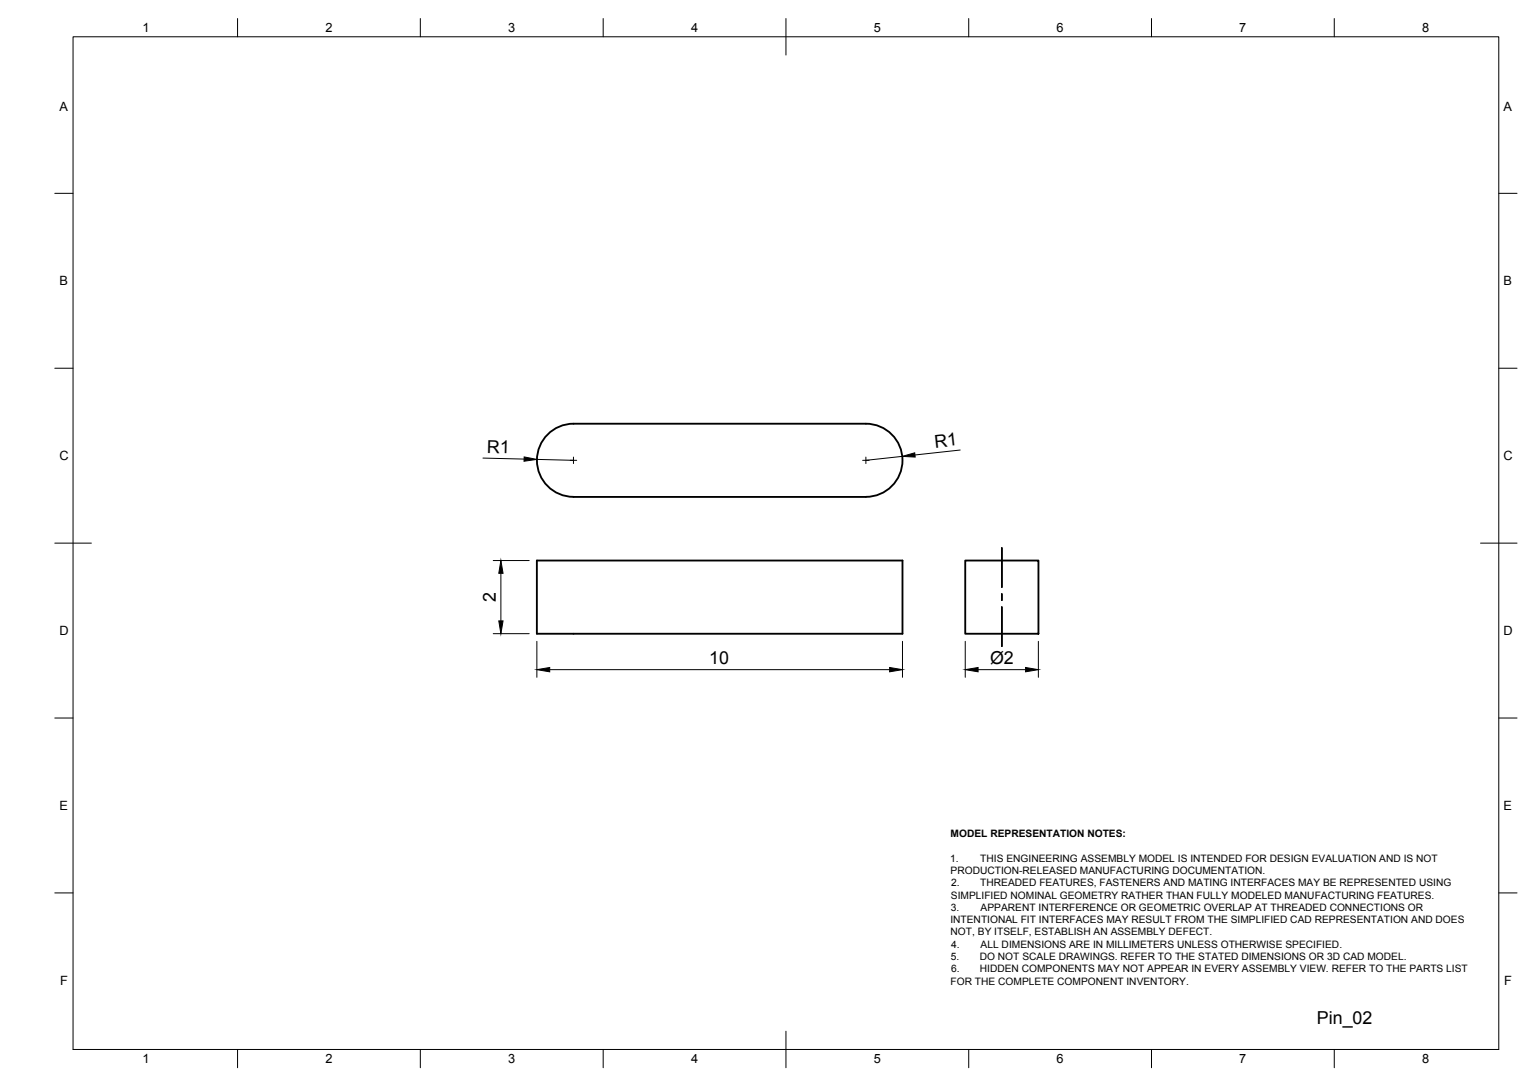
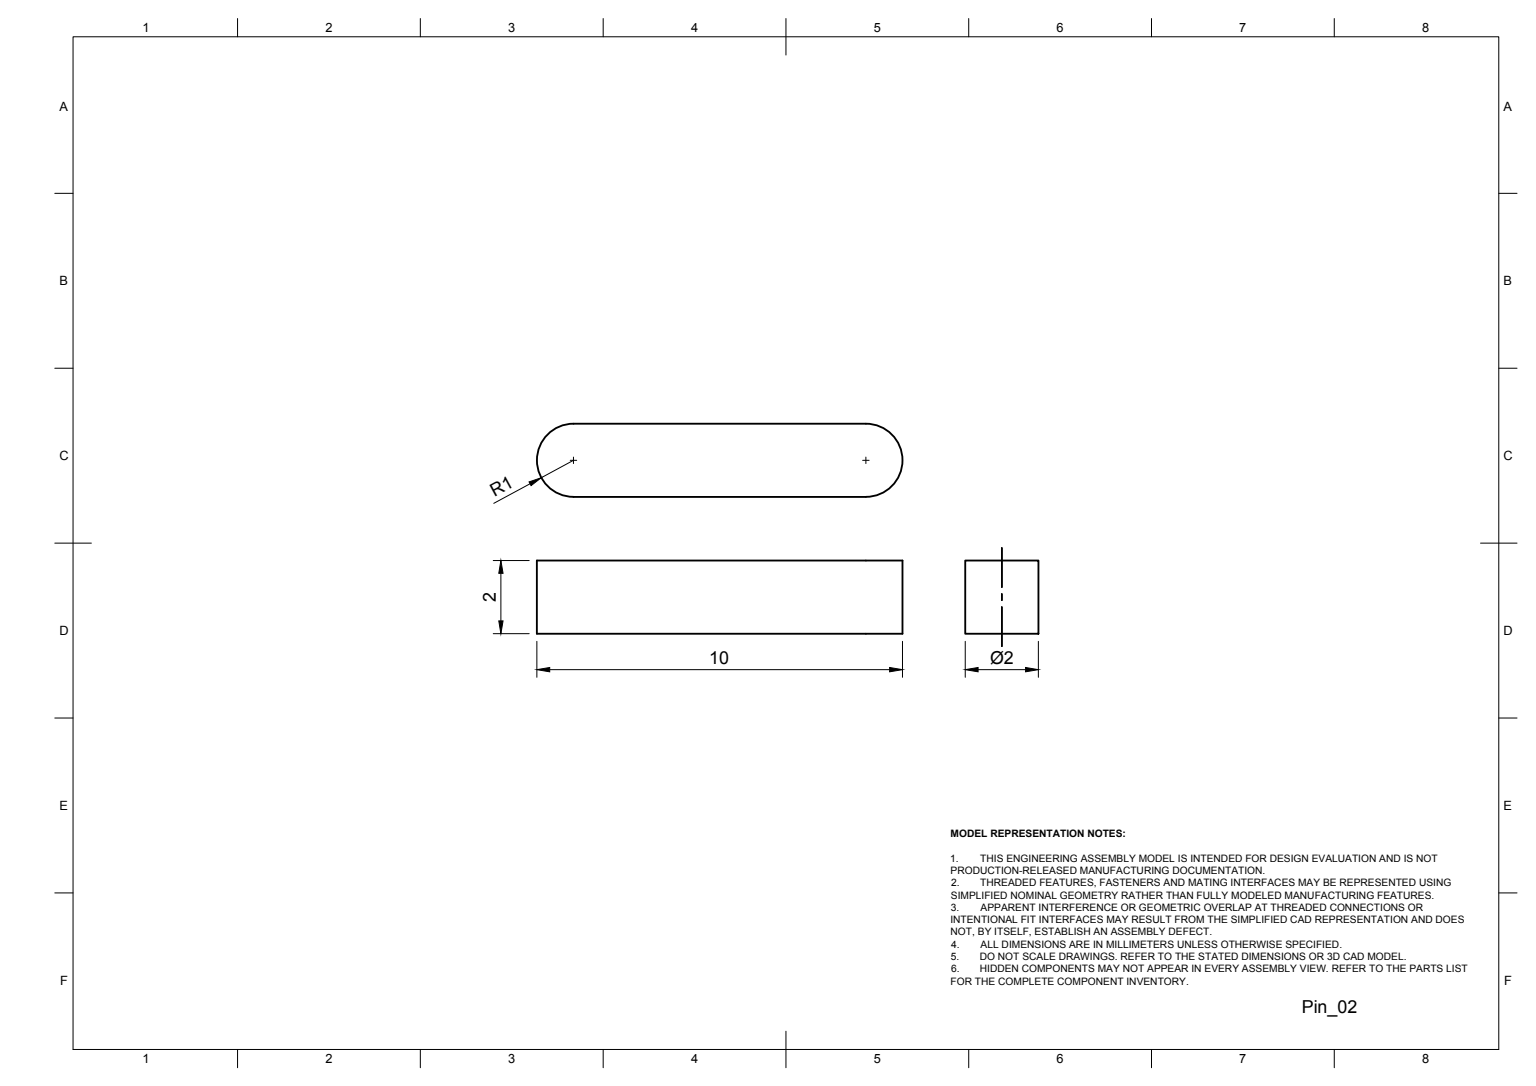
ISO-10303-21;
HEADER;
/* Generated by software containing ST-Developer
 * from STEP Tools, Inc. (www.steptools.com) 
 */

FILE_DESCRIPTION(
/* description */ (''),
/* implementation_level */ '2;1');

FILE_NAME(
/* name */ 'Pin_02.step',
/* time_stamp */ '2026-10-05T21:34:53-07:00',
/* author */ (''),
/* organization */ (''),
/* preprocessor_version */ 'ST-DEVELOPER v20.2',
/* originating_system */ 'Autodesk Translation Framework v15.15.0.0',
/* authorisation */ '');

FILE_SCHEMA (('AUTOMOTIVE_DESIGN { 1 0 10303 214 3 1 1 }'));
ENDSEC;

DATA;
#10=MECHANICAL_DESIGN_GEOMETRIC_PRESENTATION_REPRESENTATION('',(#72),#9822);
#54=SHAPE_REPRESENTATION_RELATIONSHIP('SRR','None',#9864,#63);
#63=ADVANCED_BREP_SHAPE_REPRESENTATION('',(#81),#9820);
#72=STYLED_ITEM('',(#9912),#81);
#81=MANIFOLD_SOLID_BREP('Body1',#3295);
#257=PLANE('',#3697);
#258=PLANE('',#3700);
#259=PLANE('',#3705);
#260=PLANE('',#3706);
#438=FACE_OUTER_BOUND('',#639,.T.);
#439=FACE_OUTER_BOUND('',#640,.T.);
#440=FACE_OUTER_BOUND('',#641,.T.);
#441=FACE_OUTER_BOUND('',#642,.T.);
#442=FACE_OUTER_BOUND('',#643,.T.);
#443=FACE_OUTER_BOUND('',#644,.T.);
#639=EDGE_LOOP('',(#2978,#2979,#2980,#2981));
#640=EDGE_LOOP('',(#2982,#2983,#2984,#2985));
#641=EDGE_LOOP('',(#2986,#2987,#2988,#2989));
#642=EDGE_LOOP('',(#2990,#2991,#2992,#2993));
#643=EDGE_LOOP('',(#2994,#2995,#2996,#2997));
#644=EDGE_LOOP('',(#2998,#2999,#3000,#3001));
#894=LINE('',#9744,#1153);
#895=LINE('',#9747,#1154);
#896=LINE('',#9750,#1155);
#897=LINE('',#9752,#1156);
#898=LINE('',#9753,#1157);
#899=LINE('',#9757,#1158);
#900=LINE('',#9760,#1159);
#901=LINE('',#9763,#1160);
#1153=VECTOR('',#4574,10.);
#1154=VECTOR('',#4577,10.);
#1155=VECTOR('',#4580,10.);
#1156=VECTOR('',#4581,10.);
#1157=VECTOR('',#4582,10.);
#1158=VECTOR('',#4587,10.);
#1159=VECTOR('',#4590,10.);
#1160=VECTOR('',#4595,10.);
#1311=CIRCLE('',#3698,1.);
#1312=CIRCLE('',#3699,1.);
#1313=CIRCLE('',#3702,1.);
#1314=CIRCLE('',#3704,1.);
#1609=VERTEX_POINT('',#9740);
#1610=VERTEX_POINT('',#9741);
#1611=VERTEX_POINT('',#9743);
#1612=VERTEX_POINT('',#9745);
#1613=VERTEX_POINT('',#9749);
#1614=VERTEX_POINT('',#9751);
#1615=VERTEX_POINT('',#9755);
#1616=VERTEX_POINT('',#9759);
#2068=EDGE_CURVE('',#1609,#1610,#1311,.T.);
#2069=EDGE_CURVE('',#1610,#1611,#894,.T.);
#2070=EDGE_CURVE('',#1611,#1612,#1312,.T.);
#2071=EDGE_CURVE('',#1612,#1609,#895,.T.);
#2072=EDGE_CURVE('',#1612,#1613,#896,.T.);
#2073=EDGE_CURVE('',#1613,#1614,#897,.T.);
#2074=EDGE_CURVE('',#1609,#1614,#898,.T.);
#2075=EDGE_CURVE('',#1614,#1615,#1313,.T.);
#2076=EDGE_CURVE('',#1610,#1615,#899,.T.);
#2077=EDGE_CURVE('',#1611,#1616,#900,.T.);
#2078=EDGE_CURVE('',#1616,#1613,#1314,.T.);
#2079=EDGE_CURVE('',#1615,#1616,#901,.T.);
#2978=ORIENTED_EDGE('',*,*,#2068,.T.);
#2979=ORIENTED_EDGE('',*,*,#2069,.T.);
#2980=ORIENTED_EDGE('',*,*,#2070,.T.);
#2981=ORIENTED_EDGE('',*,*,#2071,.T.);
#2982=ORIENTED_EDGE('',*,*,#2071,.F.);
#2983=ORIENTED_EDGE('',*,*,#2072,.T.);
#2984=ORIENTED_EDGE('',*,*,#2073,.T.);
#2985=ORIENTED_EDGE('',*,*,#2074,.F.);
#2986=ORIENTED_EDGE('',*,*,#2068,.F.);
#2987=ORIENTED_EDGE('',*,*,#2074,.T.);
#2988=ORIENTED_EDGE('',*,*,#2075,.T.);
#2989=ORIENTED_EDGE('',*,*,#2076,.F.);
#2990=ORIENTED_EDGE('',*,*,#2070,.F.);
#2991=ORIENTED_EDGE('',*,*,#2077,.T.);
#2992=ORIENTED_EDGE('',*,*,#2078,.T.);
#2993=ORIENTED_EDGE('',*,*,#2072,.F.);
#2994=ORIENTED_EDGE('',*,*,#2069,.F.);
#2995=ORIENTED_EDGE('',*,*,#2076,.T.);
#2996=ORIENTED_EDGE('',*,*,#2079,.T.);
#2997=ORIENTED_EDGE('',*,*,#2077,.F.);
#2998=ORIENTED_EDGE('',*,*,#2075,.F.);
#2999=ORIENTED_EDGE('',*,*,#2073,.F.);
#3000=ORIENTED_EDGE('',*,*,#2078,.F.);
#3001=ORIENTED_EDGE('',*,*,#2079,.F.);
#3099=CYLINDRICAL_SURFACE('',#3701,1.);
#3100=CYLINDRICAL_SURFACE('',#3703,1.);
#3276=ADVANCED_FACE('',(#438),#257,.F.);
#3277=ADVANCED_FACE('',(#439),#258,.F.);
#3278=ADVANCED_FACE('',(#440),#3099,.T.);
#3279=ADVANCED_FACE('',(#441),#3100,.T.);
#3280=ADVANCED_FACE('',(#442),#259,.F.);
#3281=ADVANCED_FACE('',(#443),#260,.T.);
#3295=CLOSED_SHELL('',(#3276,#3277,#3278,#3279,#3280,#3281));
#3696=AXIS2_PLACEMENT_3D('',#9738,#4568,#4569);
#3697=AXIS2_PLACEMENT_3D('',#9739,#4570,#4571);
#3698=AXIS2_PLACEMENT_3D('',#9742,#4572,#4573);
#3699=AXIS2_PLACEMENT_3D('',#9746,#4575,#4576);
#3700=AXIS2_PLACEMENT_3D('',#9748,#4578,#4579);
#3701=AXIS2_PLACEMENT_3D('',#9754,#4583,#4584);
#3702=AXIS2_PLACEMENT_3D('',#9756,#4585,#4586);
#3703=AXIS2_PLACEMENT_3D('',#9758,#4588,#4589);
#3704=AXIS2_PLACEMENT_3D('',#9761,#4591,#4592);
#3705=AXIS2_PLACEMENT_3D('',#9762,#4593,#4594);
#3706=AXIS2_PLACEMENT_3D('',#9764,#4596,#4597);
#4568=DIRECTION('axis',(0.,0.,1.));
#4569=DIRECTION('refdir',(1.,0.,0.));
#4570=DIRECTION('center_axis',(0.,-1.,0.));
#4571=DIRECTION('ref_axis',(1.,0.,0.));
#4572=DIRECTION('center_axis',(0.,1.,0.));
#4573=DIRECTION('ref_axis',(1.,0.,0.));
#4574=DIRECTION('',(0.,0.,-1.));
#4575=DIRECTION('center_axis',(0.,1.,0.));
#4576=DIRECTION('ref_axis',(-1.,0.,0.));
#4577=DIRECTION('',(0.,0.,1.));
#4578=DIRECTION('center_axis',(1.,0.,0.));
#4579=DIRECTION('ref_axis',(0.,0.,1.));
#4580=DIRECTION('',(0.,-1.,0.));
#4581=DIRECTION('',(0.,0.,1.));
#4582=DIRECTION('',(0.,-1.,0.));
#4583=DIRECTION('center_axis',(0.,1.,0.));
#4584=DIRECTION('ref_axis',(1.,0.,0.));
#4585=DIRECTION('center_axis',(0.,1.,0.));
#4586=DIRECTION('ref_axis',(1.,0.,0.));
#4587=DIRECTION('',(0.,-1.,0.));
#4588=DIRECTION('center_axis',(0.,1.,0.));
#4589=DIRECTION('ref_axis',(-1.,0.,0.));
#4590=DIRECTION('',(0.,-1.,0.));
#4591=DIRECTION('center_axis',(0.,1.,0.));
#4592=DIRECTION('ref_axis',(-1.,0.,0.));
#4593=DIRECTION('center_axis',(-1.,0.,0.));
#4594=DIRECTION('ref_axis',(0.,0.,-1.));
#4595=DIRECTION('',(0.,0.,-1.));
#4596=DIRECTION('center_axis',(0.,-1.,0.));
#4597=DIRECTION('ref_axis',(1.,0.,0.));
#9738=CARTESIAN_POINT('',(0.,0.,0.));
#9739=CARTESIAN_POINT('Origin',(0.,-4.,-10.5));
#9740=CARTESIAN_POINT('',(-1.,-4.,-6.5));
#9741=CARTESIAN_POINT('',(1.,-4.,-6.5));
#9742=CARTESIAN_POINT('Origin',(0.,-4.,-6.5));
#9743=CARTESIAN_POINT('',(1.,-4.,-14.5));
#9744=CARTESIAN_POINT('',(1.,-4.,-8.5));
#9745=CARTESIAN_POINT('',(-1.,-4.,-14.5));
#9746=CARTESIAN_POINT('Origin',(0.,-4.,-14.5));
#9747=CARTESIAN_POINT('',(-1.,-4.,-12.5));
#9748=CARTESIAN_POINT('Origin',(-1.,0.,-14.5));
#9749=CARTESIAN_POINT('',(-1.,-6.,-14.5));
#9750=CARTESIAN_POINT('',(-1.,0.,-14.5));
#9751=CARTESIAN_POINT('',(-1.,-6.,-6.5));
#9752=CARTESIAN_POINT('',(-1.,-6.,-6.5));
#9753=CARTESIAN_POINT('',(-1.,0.,-6.5));
#9754=CARTESIAN_POINT('Origin',(0.,0.,-6.5));
#9755=CARTESIAN_POINT('',(1.,-6.,-6.5));
#9756=CARTESIAN_POINT('Origin',(0.,-6.,-6.5));
#9757=CARTESIAN_POINT('',(1.,0.,-6.5));
#9758=CARTESIAN_POINT('Origin',(0.,0.,-14.5));
#9759=CARTESIAN_POINT('',(1.,-6.,-14.5));
#9760=CARTESIAN_POINT('',(1.,0.,-14.5));
#9761=CARTESIAN_POINT('Origin',(0.,-6.,-14.5));
#9762=CARTESIAN_POINT('Origin',(1.,0.,-6.5));
#9763=CARTESIAN_POINT('',(1.,-6.,-14.5));
#9764=CARTESIAN_POINT('Origin',(0.,-6.,-10.5));
#9809=UNCERTAINTY_MEASURE_WITH_UNIT(LENGTH_MEASURE(0.01),#9823,
'DISTANCE_ACCURACY_VALUE',
'Maximum model space distance between geometric entities at asserted c
onnectivities');
#9811=UNCERTAINTY_MEASURE_WITH_UNIT(LENGTH_MEASURE(0.01),#9823,
'DISTANCE_ACCURACY_VALUE',
'Maximum model space distance between geometric entities at asserted c
onnectivities');
#9820=(
GEOMETRIC_REPRESENTATION_CONTEXT(3)
GLOBAL_UNCERTAINTY_ASSIGNED_CONTEXT((#9809))
GLOBAL_UNIT_ASSIGNED_CONTEXT((#9823,#9825,#9826))
REPRESENTATION_CONTEXT('','3D')
);
#9822=(
GEOMETRIC_REPRESENTATION_CONTEXT(3)
GLOBAL_UNCERTAINTY_ASSIGNED_CONTEXT((#9811))
GLOBAL_UNIT_ASSIGNED_CONTEXT((#9823,#9825,#9826))
REPRESENTATION_CONTEXT('','3D')
);
#9823=(
LENGTH_UNIT()
NAMED_UNIT(*)
SI_UNIT(.MILLI.,.METRE.)
);
#9825=(
NAMED_UNIT(*)
PLANE_ANGLE_UNIT()
SI_UNIT($,.RADIAN.)
);
#9826=(
NAMED_UNIT(*)
SI_UNIT($,.STERADIAN.)
SOLID_ANGLE_UNIT()
);
#9835=SHAPE_DEFINITION_REPRESENTATION(#9845,#9864);
#9845=PRODUCT_DEFINITION_SHAPE('',$,#9875);
#9864=SHAPE_REPRESENTATION('',(#3696),#9820);
#9866=PRODUCT_DEFINITION_CONTEXT('part definition',#9898,'design');
#9875=PRODUCT_DEFINITION('Pin_02','Pin_02',#9885,#9866);
#9885=PRODUCT_DEFINITION_FORMATION('',$,#9908);
#9898=APPLICATION_CONTEXT(
'Core Data for Automotive Mechanical Design Process');
#9899=PRODUCT_CONTEXT('part definition',#9898,'mechanical');
#9908=PRODUCT('Pin_02','Pin_02',$,(#9899));
#9912=PRESENTATION_STYLE_ASSIGNMENT((#9915));
#9915=SURFACE_STYLE_USAGE(.BOTH.,#9918);
#9918=SURFACE_SIDE_STYLE('',(#9921));
#9921=SURFACE_STYLE_FILL_AREA(#9924);
#9924=FILL_AREA_STYLE('Opaque(233,233,233)',(#9927));
#9927=FILL_AREA_STYLE_COLOUR('Opaque(233,233,233)',#9930);
#9930=COLOUR_RGB('Opaque(233,233,233)', 0.40784314, 0.44705882, 0.49803922);
ENDSEC;
END-ISO-10303-21;
